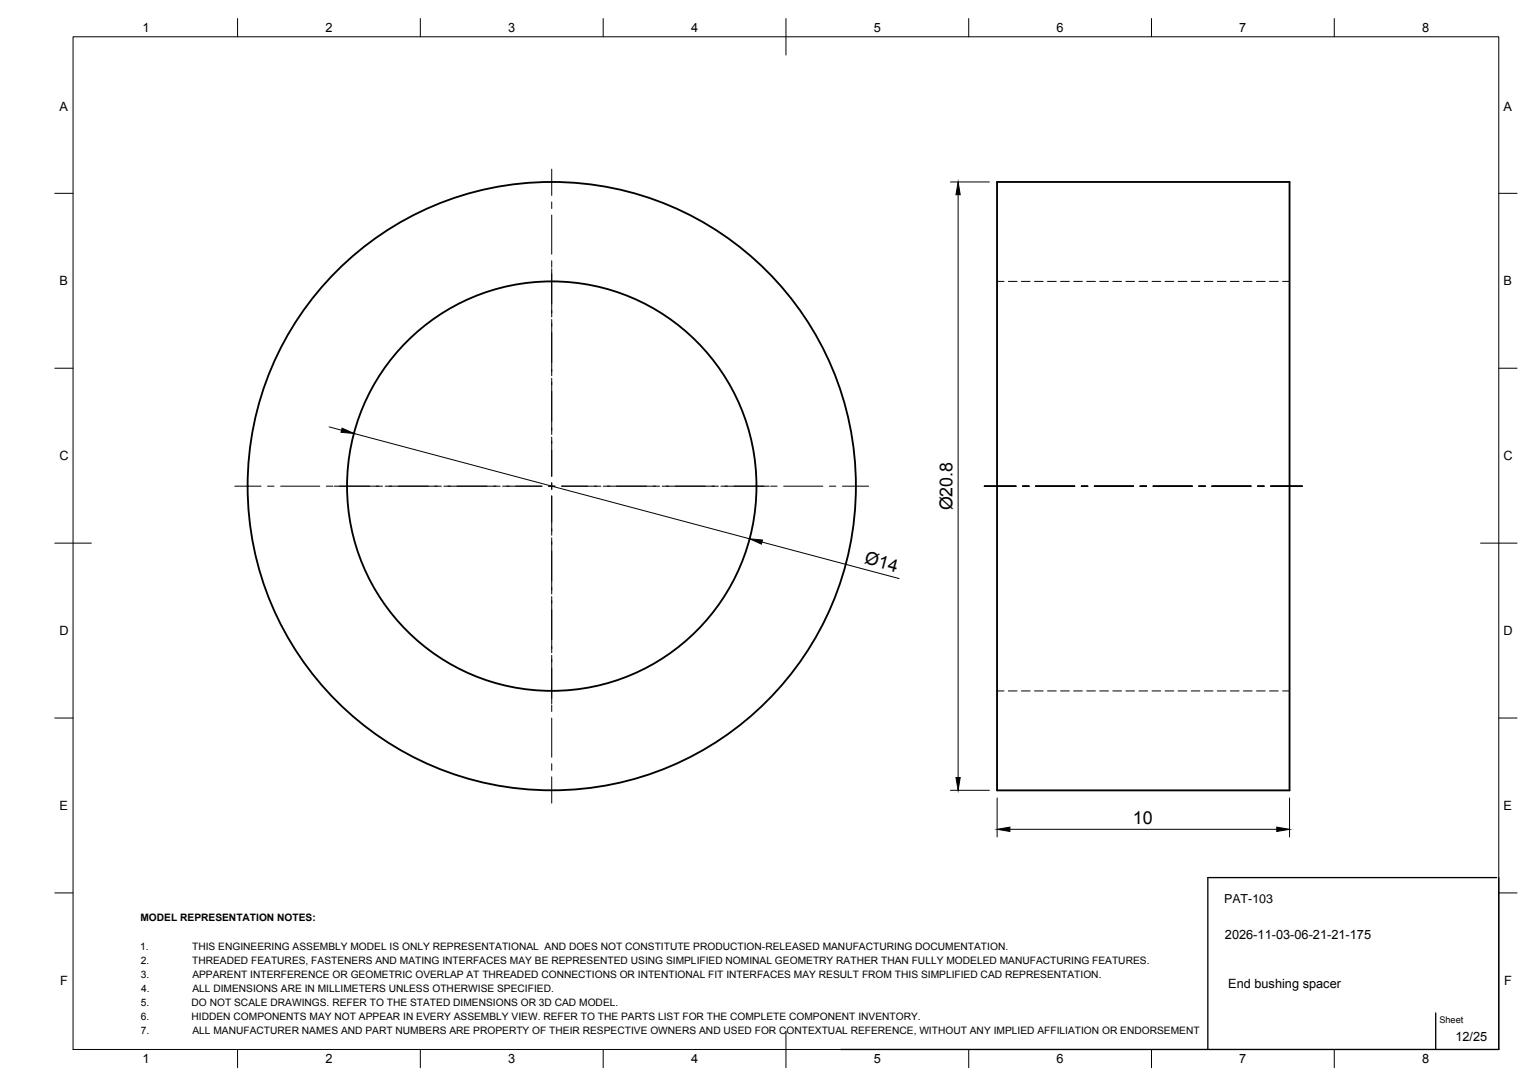
ISO-10303-21;
HEADER;
/* Generated by software containing ST-Developer
 * from STEP Tools, Inc. (www.steptools.com) 
 */

FILE_DESCRIPTION(
/* description */ ('Telescoping shaft support with lock collar'),
/* implementation_level */ '2;1');

FILE_NAME(
/* name */ 'End bushing spacer.step',
/* time_stamp */ '2026-10-27T10:48:51-07:00',
/* author */ (''),
/* organization */ (''),
/* preprocessor_version */ 'ST-DEVELOPER v20.2',
/* originating_system */ 'Autodesk Translation Framework v15.17.0.0',
/* authorisation */ '');

FILE_SCHEMA (('AUTOMOTIVE_DESIGN { 1 0 10303 214 3 1 1 }'));
ENDSEC;

DATA;
#10=MECHANICAL_DESIGN_GEOMETRIC_PRESENTATION_REPRESENTATION('',(#248),#7349);
#208=SHAPE_REPRESENTATION_RELATIONSHIP('SRR','None',#7450,#228);
#228=ADVANCED_BREP_SHAPE_REPRESENTATION('',(#268),#7334);
#248=STYLED_ITEM('',(#7641),#268);
#268=MANIFOLD_SOLID_BREP('Body1',#3971);
#315=FACE_BOUND('',#854,.T.);
#316=FACE_BOUND('',#856,.T.);
#417=PLANE('',#4413);
#418=PLANE('',#4414);
#589=FACE_OUTER_BOUND('',#851,.T.);
#590=FACE_OUTER_BOUND('',#852,.T.);
#591=FACE_OUTER_BOUND('',#853,.T.);
#592=FACE_OUTER_BOUND('',#855,.T.);
#851=EDGE_LOOP('',(#3098,#3099,#3100,#3101));
#852=EDGE_LOOP('',(#3102,#3103,#3104,#3105));
#853=EDGE_LOOP('',(#3106));
#854=EDGE_LOOP('',(#3107));
#855=EDGE_LOOP('',(#3108));
#856=EDGE_LOOP('',(#3109));
#1159=LINE('',#6475,#1439);
#1160=LINE('',#6481,#1440);
#1439=VECTOR('',#5243,0.7);
#1440=VECTOR('',#5250,1.04);
#1683=CIRCLE('',#4408,0.7);
#1684=CIRCLE('',#4409,0.7);
#1685=CIRCLE('',#4411,1.04);
#1686=CIRCLE('',#4412,1.04);
#1950=VERTEX_POINT('',#6472);
#1951=VERTEX_POINT('',#6474);
#1952=VERTEX_POINT('',#6478);
#1953=VERTEX_POINT('',#6480);
#2361=EDGE_CURVE('',#1950,#1950,#1683,.T.);
#2362=EDGE_CURVE('',#1950,#1951,#1159,.T.);
#2363=EDGE_CURVE('',#1951,#1951,#1684,.T.);
#2364=EDGE_CURVE('',#1952,#1952,#1685,.T.);
#2365=EDGE_CURVE('',#1952,#1953,#1160,.T.);
#2366=EDGE_CURVE('',#1953,#1953,#1686,.T.);
#3098=ORIENTED_EDGE('',*,*,#2361,.F.);
#3099=ORIENTED_EDGE('',*,*,#2362,.T.);
#3100=ORIENTED_EDGE('',*,*,#2363,.T.);
#3101=ORIENTED_EDGE('',*,*,#2362,.F.);
#3102=ORIENTED_EDGE('',*,*,#2364,.F.);
#3103=ORIENTED_EDGE('',*,*,#2365,.T.);
#3104=ORIENTED_EDGE('',*,*,#2366,.T.);
#3105=ORIENTED_EDGE('',*,*,#2365,.F.);
#3106=ORIENTED_EDGE('',*,*,#2364,.T.);
#3107=ORIENTED_EDGE('',*,*,#2361,.T.);
#3108=ORIENTED_EDGE('',*,*,#2366,.F.);
#3109=ORIENTED_EDGE('',*,*,#2363,.F.);
#3696=CYLINDRICAL_SURFACE('',#4407,0.7);
#3697=CYLINDRICAL_SURFACE('',#4410,1.04);
#3832=ADVANCED_FACE('',(#589),#3696,.F.);
#3833=ADVANCED_FACE('',(#590),#3697,.T.);
#3834=ADVANCED_FACE('',(#591,#315),#417,.T.);
#3835=ADVANCED_FACE('',(#592,#316),#418,.F.);
#3971=CLOSED_SHELL('',(#3832,#3833,#3834,#3835));
#4406=AXIS2_PLACEMENT_3D('',#6470,#5237,#5238);
#4407=AXIS2_PLACEMENT_3D('',#6471,#5239,#5240);
#4408=AXIS2_PLACEMENT_3D('',#6473,#5241,#5242);
#4409=AXIS2_PLACEMENT_3D('',#6476,#5244,#5245);
#4410=AXIS2_PLACEMENT_3D('',#6477,#5246,#5247);
#4411=AXIS2_PLACEMENT_3D('',#6479,#5248,#5249);
#4412=AXIS2_PLACEMENT_3D('',#6482,#5251,#5252);
#4413=AXIS2_PLACEMENT_3D('',#6483,#5253,#5254);
#4414=AXIS2_PLACEMENT_3D('',#6484,#5255,#5256);
#5237=DIRECTION('axis',(0.,0.,1.));
#5238=DIRECTION('refdir',(1.,0.,0.));
#5239=DIRECTION('center_axis',(1.,0.,0.));
#5240=DIRECTION('ref_axis',(0.,0.,-1.));
#5241=DIRECTION('center_axis',(-1.,0.,0.));
#5242=DIRECTION('ref_axis',(0.,0.,-1.));
#5243=DIRECTION('',(-1.,0.,0.));
#5244=DIRECTION('center_axis',(-1.,0.,0.));
#5245=DIRECTION('ref_axis',(0.,0.,-1.));
#5246=DIRECTION('center_axis',(1.,0.,0.));
#5247=DIRECTION('ref_axis',(0.,0.,-1.));
#5248=DIRECTION('center_axis',(1.,0.,0.));
#5249=DIRECTION('ref_axis',(0.,0.,-1.));
#5250=DIRECTION('',(-1.,0.,0.));
#5251=DIRECTION('center_axis',(1.,0.,0.));
#5252=DIRECTION('ref_axis',(0.,0.,-1.));
#5253=DIRECTION('center_axis',(1.,0.,0.));
#5254=DIRECTION('ref_axis',(0.,0.,-1.));
#5255=DIRECTION('center_axis',(1.,0.,0.));
#5256=DIRECTION('ref_axis',(0.,0.,-1.));
#6470=CARTESIAN_POINT('',(0.,0.,0.));
#6471=CARTESIAN_POINT('Origin',(0.,0.,3.5));
#6472=CARTESIAN_POINT('',(1.,-8.57252759403147E-17,4.2));
#6473=CARTESIAN_POINT('Origin',(1.,0.,3.5));
#6474=CARTESIAN_POINT('',(0.,-8.57252759403147E-17,4.2));
#6475=CARTESIAN_POINT('',(0.,-8.57252759403147E-17,4.2));
#6476=CARTESIAN_POINT('Origin',(0.,0.,3.5));
#6477=CARTESIAN_POINT('Origin',(0.,0.,3.5));
#6478=CARTESIAN_POINT('',(1.,-1.27363267111325E-16,4.54));
#6479=CARTESIAN_POINT('Origin',(1.,0.,3.5));
#6480=CARTESIAN_POINT('',(0.,-1.27363267111325E-16,4.54));
#6481=CARTESIAN_POINT('',(0.,-1.27363267111325E-16,4.54));
#6482=CARTESIAN_POINT('Origin',(0.,0.,3.5));
#6483=CARTESIAN_POINT('Origin',(1.,0.,3.5));
#6484=CARTESIAN_POINT('Origin',(0.,0.,3.5));
#7309=UNCERTAINTY_MEASURE_WITH_UNIT(LENGTH_MEASURE(0.001),#7350,
'DISTANCE_ACCURACY_VALUE',
'Maximum model space distance between geometric entities at asserted c
onnectivities');
#7324=UNCERTAINTY_MEASURE_WITH_UNIT(LENGTH_MEASURE(0.001),#7350,
'DISTANCE_ACCURACY_VALUE',
'Maximum model space distance between geometric entities at asserted c
onnectivities');
#7334=(
GEOMETRIC_REPRESENTATION_CONTEXT(3)
GLOBAL_UNCERTAINTY_ASSIGNED_CONTEXT((#7309))
GLOBAL_UNIT_ASSIGNED_CONTEXT((#7350,#7352,#7353))
REPRESENTATION_CONTEXT('','3D')
);
#7349=(
GEOMETRIC_REPRESENTATION_CONTEXT(3)
GLOBAL_UNCERTAINTY_ASSIGNED_CONTEXT((#7324))
GLOBAL_UNIT_ASSIGNED_CONTEXT((#7350,#7352,#7353))
REPRESENTATION_CONTEXT('','3D')
);
#7350=(
LENGTH_UNIT()
NAMED_UNIT(*)
SI_UNIT(.CENTI.,.METRE.)
);
#7352=(
NAMED_UNIT(*)
PLANE_ANGLE_UNIT()
SI_UNIT($,.RADIAN.)
);
#7353=(
NAMED_UNIT(*)
SI_UNIT($,.STERADIAN.)
SOLID_ANGLE_UNIT()
);
#7363=SHAPE_DEFINITION_REPRESENTATION(#7387,#7450);
#7387=PRODUCT_DEFINITION_SHAPE('',$,#7475);
#7450=SHAPE_REPRESENTATION('',(#4406),#7334);
#7465=PRODUCT_DEFINITION_CONTEXT('part definition',#7539,'design');
#7475=PRODUCT_DEFINITION('End bushing spacer','End bushing spacer',#7499,
#7465);
#7499=PRODUCT_DEFINITION_FORMATION('',$,#7550);
#7539=APPLICATION_CONTEXT(
'Core Data for Automotive Mechanical Design Process');
#7540=PRODUCT_CONTEXT('part definition',#7539,'mechanical');
#7550=PRODUCT('End bushing spacer','End bushing spacer',
'End bushing spacer',(#7540));
#7635=COLOUR_RGB('Off White',0.89,0.88,0.83);
#7636=FILL_AREA_STYLE_COLOUR('',#7635);
#7637=FILL_AREA_STYLE('',(#7636));
#7638=SURFACE_STYLE_FILL_AREA(#7637);
#7639=SURFACE_SIDE_STYLE('',(#7638));
#7640=SURFACE_STYLE_USAGE(.BOTH.,#7639);
#7641=PRESENTATION_STYLE_ASSIGNMENT((#7640));
ENDSEC;
END-ISO-10303-21;
